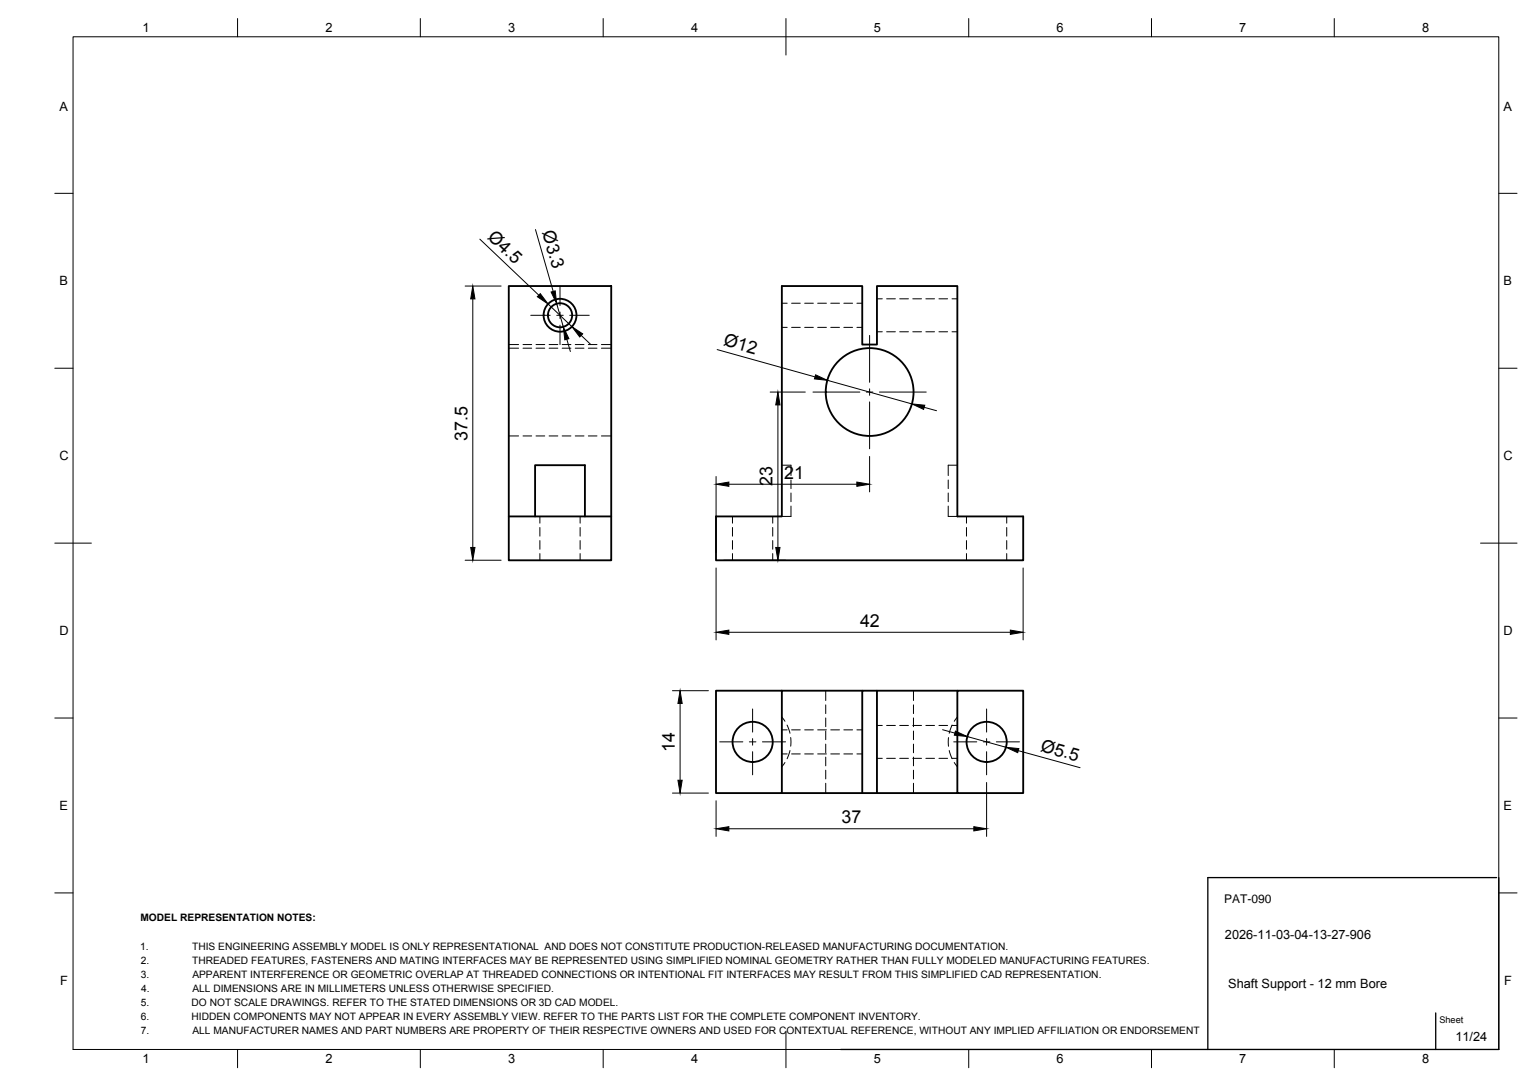
ISO-10303-21;
HEADER;
/* Generated by software containing ST-Developer
 * from STEP Tools, Inc. (www.steptools.com) 
 */

FILE_DESCRIPTION(
/* description */ ('Round-Shaft Linear Stage with Ball Bushings'),
/* implementation_level */ '2;1');

FILE_NAME(
/* name */ 'Shaft Support - 12 mm Bore.step',
/* time_stamp */ '2026-10-27T10:47:55-07:00',
/* author */ (''),
/* organization */ (''),
/* preprocessor_version */ 'ST-DEVELOPER v20.2',
/* originating_system */ 'Autodesk Translation Framework v15.17.0.0',
/* authorisation */ '');

FILE_SCHEMA (('AUTOMOTIVE_DESIGN { 1 0 10303 214 3 1 1 }'));
ENDSEC;

DATA;
#10=MECHANICAL_DESIGN_GEOMETRIC_PRESENTATION_REPRESENTATION('',(#308),#7835);
#266=SHAPE_REPRESENTATION_RELATIONSHIP('SRR','None',#7954,#287);
#287=ADVANCED_BREP_SHAPE_REPRESENTATION('',(#329),#7818);
#308=STYLED_ITEM('',(#8144),#329);
#329=MANIFOLD_SOLID_BREP('Body1',#4398);
#376=FACE_BOUND('',#973,.T.);
#377=FACE_BOUND('',#975,.T.);
#378=FACE_BOUND('',#977,.T.);
#379=FACE_BOUND('',#984,.T.);
#380=FACE_BOUND('',#987,.T.);
#381=FACE_BOUND('',#988,.T.);
#382=FACE_BOUND('',#991,.T.);
#383=FACE_BOUND('',#994,.T.);
#384=FACE_BOUND('',#997,.T.);
#385=FACE_BOUND('',#1000,.T.);
#495=PLANE('',#4761);
#496=PLANE('',#4768);
#497=PLANE('',#4769);
#498=PLANE('',#4771);
#499=PLANE('',#4773);
#500=PLANE('',#4787);
#501=PLANE('',#4788);
#502=PLANE('',#4789);
#503=PLANE('',#4790);
#504=PLANE('',#4791);
#505=PLANE('',#4792);
#506=PLANE('',#4793);
#507=PLANE('',#4794);
#508=PLANE('',#4795);
#509=PLANE('',#4796);
#510=PLANE('',#4797);
#675=FACE_OUTER_BOUND('',#968,.T.);
#676=FACE_OUTER_BOUND('',#969,.T.);
#677=FACE_OUTER_BOUND('',#970,.T.);
#678=FACE_OUTER_BOUND('',#971,.T.);
#679=FACE_OUTER_BOUND('',#972,.T.);
#680=FACE_OUTER_BOUND('',#974,.T.);
#681=FACE_OUTER_BOUND('',#976,.T.);
#682=FACE_OUTER_BOUND('',#978,.T.);
#683=FACE_OUTER_BOUND('',#979,.T.);
#684=FACE_OUTER_BOUND('',#980,.T.);
#685=FACE_OUTER_BOUND('',#981,.T.);
#686=FACE_OUTER_BOUND('',#982,.T.);
#687=FACE_OUTER_BOUND('',#983,.T.);
#688=FACE_OUTER_BOUND('',#985,.T.);
#689=FACE_OUTER_BOUND('',#986,.T.);
#690=FACE_OUTER_BOUND('',#989,.T.);
#691=FACE_OUTER_BOUND('',#990,.T.);
#692=FACE_OUTER_BOUND('',#992,.T.);
#693=FACE_OUTER_BOUND('',#993,.T.);
#694=FACE_OUTER_BOUND('',#995,.T.);
#695=FACE_OUTER_BOUND('',#996,.T.);
#696=FACE_OUTER_BOUND('',#998,.T.);
#697=FACE_OUTER_BOUND('',#999,.T.);
#968=EDGE_LOOP('',(#3248,#3249));
#969=EDGE_LOOP('',(#3250,#3251,#3252,#3253));
#970=EDGE_LOOP('',(#3254,#3255,#3256,#3257));
#971=EDGE_LOOP('',(#3258,#3259));
#972=EDGE_LOOP('',(#3260,#3261,#3262,#3263,#3264,#3265));
#973=EDGE_LOOP('',(#3266));
#974=EDGE_LOOP('',(#3267,#3268,#3269,#3270,#3271,#3272,#3273,#3274));
#975=EDGE_LOOP('',(#3275));
#976=EDGE_LOOP('',(#3276,#3277,#3278,#3279,#3280,#3281));
#977=EDGE_LOOP('',(#3282));
#978=EDGE_LOOP('',(#3283,#3284,#3285,#3286));
#979=EDGE_LOOP('',(#3287,#3288,#3289,#3290));
#980=EDGE_LOOP('',(#3291,#3292,#3293,#3294));
#981=EDGE_LOOP('',(#3295,#3296,#3297,#3298));
#982=EDGE_LOOP('',(#3299,#3300,#3301,#3302));
#983=EDGE_LOOP('',(#3303,#3304,#3305,#3306,#3307,#3308,#3309,#3310,#3311,
#3312,#3313,#3314));
#984=EDGE_LOOP('',(#3315));
#985=EDGE_LOOP('',(#3316,#3317,#3318,#3319));
#986=EDGE_LOOP('',(#3320,#3321,#3322,#3323));
#987=EDGE_LOOP('',(#3324));
#988=EDGE_LOOP('',(#3325));
#989=EDGE_LOOP('',(#3326,#3327,#3328,#3329));
#990=EDGE_LOOP('',(#3330,#3331,#3332,#3333,#3334,#3335,#3336,#3337));
#991=EDGE_LOOP('',(#3338));
#992=EDGE_LOOP('',(#3339,#3340,#3341,#3342));
#993=EDGE_LOOP('',(#3343,#3344,#3345,#3346));
#994=EDGE_LOOP('',(#3347));
#995=EDGE_LOOP('',(#3348,#3349,#3350,#3351));
#996=EDGE_LOOP('',(#3352,#3353,#3354,#3355));
#997=EDGE_LOOP('',(#3356));
#998=EDGE_LOOP('',(#3357,#3358,#3359,#3360));
#999=EDGE_LOOP('',(#3361,#3362,#3363,#3364,#3365,#3366,#3367,#3368,#3369,
#3370,#3371,#3372));
#1000=EDGE_LOOP('',(#3373));
#1332=LINE('',#6852,#1672);
#1333=LINE('',#6856,#1673);
#1334=LINE('',#6859,#1674);
#1335=LINE('',#6863,#1675);
#1336=LINE('',#6867,#1676);
#1337=LINE('',#6870,#1677);
#1338=LINE('',#6873,#1678);
#1339=LINE('',#6875,#1679);
#1340=LINE('',#6877,#1680);
#1341=LINE('',#6879,#1681);
#1342=LINE('',#6880,#1682);
#1343=LINE('',#6885,#1683);
#1344=LINE('',#6887,#1684);
#1345=LINE('',#6888,#1685);
#1346=LINE('',#6894,#1686);
#1347=LINE('',#6896,#1687);
#1348=LINE('',#6897,#1688);
#1349=LINE('',#6899,#1689);
#1350=LINE('',#6900,#1690);
#1351=LINE('',#6907,#1691);
#1352=LINE('',#6911,#1692);
#1353=LINE('',#6916,#1693);
#1354=LINE('',#6920,#1694);
#1355=LINE('',#6925,#1695);
#1356=LINE('',#6929,#1696);
#1357=LINE('',#6931,#1697);
#1358=LINE('',#6932,#1698);
#1359=LINE('',#6934,#1699);
#1360=LINE('',#6936,#1700);
#1361=LINE('',#6938,#1701);
#1362=LINE('',#6940,#1702);
#1363=LINE('',#6942,#1703);
#1364=LINE('',#6943,#1704);
#1365=LINE('',#6946,#1705);
#1366=LINE('',#6947,#1706);
#1367=LINE('',#6950,#1707);
#1368=LINE('',#6951,#1708);
#1369=LINE('',#6953,#1709);
#1370=LINE('',#6956,#1710);
#1371=LINE('',#6957,#1711);
#1372=LINE('',#6960,#1712);
#1373=LINE('',#6961,#1713);
#1374=LINE('',#6964,#1714);
#1375=LINE('',#6965,#1715);
#1376=LINE('',#6968,#1716);
#1377=LINE('',#6969,#1717);
#1378=LINE('',#6972,#1718);
#1379=LINE('',#6973,#1719);
#1380=LINE('',#6975,#1720);
#1672=VECTOR('',#5485,1.);
#1673=VECTOR('',#5490,1.);
#1674=VECTOR('',#5493,1.);
#1675=VECTOR('',#5496,1.);
#1676=VECTOR('',#5499,1.);
#1677=VECTOR('',#5504,1.);
#1678=VECTOR('',#5507,1.);
#1679=VECTOR('',#5508,1.);
#1680=VECTOR('',#5509,1.);
#1681=VECTOR('',#5510,1.);
#1682=VECTOR('',#5511,1.);
#1683=VECTOR('',#5516,1.);
#1684=VECTOR('',#5517,1.);
#1685=VECTOR('',#5518,1.);
#1686=VECTOR('',#5523,1.);
#1687=VECTOR('',#5524,1.);
#1688=VECTOR('',#5525,1.);
#1689=VECTOR('',#5526,1.);
#1690=VECTOR('',#5527,1.);
#1691=VECTOR('',#5534,0.225);
#1692=VECTOR('',#5539,0.165);
#1693=VECTOR('',#5546,0.275);
#1694=VECTOR('',#5551,0.275);
#1695=VECTOR('',#5556,0.6);
#1696=VECTOR('',#5561,1.);
#1697=VECTOR('',#5562,1.);
#1698=VECTOR('',#5563,1.);
#1699=VECTOR('',#5564,1.);
#1700=VECTOR('',#5565,1.);
#1701=VECTOR('',#5566,1.);
#1702=VECTOR('',#5567,1.);
#1703=VECTOR('',#5568,1.);
#1704=VECTOR('',#5569,1.);
#1705=VECTOR('',#5572,1.);
#1706=VECTOR('',#5573,1.);
#1707=VECTOR('',#5576,1.);
#1708=VECTOR('',#5577,1.);
#1709=VECTOR('',#5580,1.);
#1710=VECTOR('',#5583,1.);
#1711=VECTOR('',#5584,1.);
#1712=VECTOR('',#5587,1.);
#1713=VECTOR('',#5588,1.);
#1714=VECTOR('',#5591,1.);
#1715=VECTOR('',#5592,1.);
#1716=VECTOR('',#5595,1.);
#1717=VECTOR('',#5596,1.);
#1718=VECTOR('',#5599,1.);
#1719=VECTOR('',#5600,1.);
#1720=VECTOR('',#5603,1.);
#1973=CIRCLE('',#4762,0.525);
#1974=CIRCLE('',#4764,0.525);
#1975=CIRCLE('',#4766,0.525);
#1976=CIRCLE('',#4767,0.525);
#1977=CIRCLE('',#4770,0.275);
#1978=CIRCLE('',#4772,0.165);
#1979=CIRCLE('',#4774,0.275);
#1980=CIRCLE('',#4776,0.225);
#1981=CIRCLE('',#4777,0.225);
#1982=CIRCLE('',#4779,0.165);
#1983=CIRCLE('',#4781,0.275);
#1984=CIRCLE('',#4783,0.275);
#1985=CIRCLE('',#4785,0.6);
#1986=CIRCLE('',#4786,0.6);
#2202=VERTEX_POINT('',#6850);
#2203=VERTEX_POINT('',#6851);
#2204=VERTEX_POINT('',#6855);
#2205=VERTEX_POINT('',#6857);
#2206=VERTEX_POINT('',#6861);
#2207=VERTEX_POINT('',#6862);
#2208=VERTEX_POINT('',#6864);
#2209=VERTEX_POINT('',#6866);
#2210=VERTEX_POINT('',#6872);
#2211=VERTEX_POINT('',#6874);
#2212=VERTEX_POINT('',#6876);
#2213=VERTEX_POINT('',#6878);
#2214=VERTEX_POINT('',#6881);
#2215=VERTEX_POINT('',#6884);
#2216=VERTEX_POINT('',#6886);
#2217=VERTEX_POINT('',#6889);
#2218=VERTEX_POINT('',#6892);
#2219=VERTEX_POINT('',#6893);
#2220=VERTEX_POINT('',#6895);
#2221=VERTEX_POINT('',#6898);
#2222=VERTEX_POINT('',#6901);
#2223=VERTEX_POINT('',#6904);
#2224=VERTEX_POINT('',#6906);
#2225=VERTEX_POINT('',#6910);
#2226=VERTEX_POINT('',#6914);
#2227=VERTEX_POINT('',#6918);
#2228=VERTEX_POINT('',#6922);
#2229=VERTEX_POINT('',#6924);
#2230=VERTEX_POINT('',#6928);
#2231=VERTEX_POINT('',#6930);
#2232=VERTEX_POINT('',#6933);
#2233=VERTEX_POINT('',#6935);
#2234=VERTEX_POINT('',#6937);
#2235=VERTEX_POINT('',#6939);
#2236=VERTEX_POINT('',#6941);
#2237=VERTEX_POINT('',#6945);
#2238=VERTEX_POINT('',#6949);
#2239=VERTEX_POINT('',#6955);
#2240=VERTEX_POINT('',#6959);
#2241=VERTEX_POINT('',#6963);
#2242=VERTEX_POINT('',#6967);
#2243=VERTEX_POINT('',#6971);
#2592=EDGE_CURVE('',#2202,#2203,#1332,.T.);
#2593=EDGE_CURVE('',#2203,#2202,#1973,.T.);
#2594=EDGE_CURVE('',#2204,#2202,#1333,.T.);
#2595=EDGE_CURVE('',#2205,#2204,#1974,.T.);
#2596=EDGE_CURVE('',#2203,#2205,#1334,.T.);
#2597=EDGE_CURVE('',#2206,#2207,#1335,.T.);
#2598=EDGE_CURVE('',#2206,#2208,#1975,.T.);
#2599=EDGE_CURVE('',#2209,#2208,#1336,.T.);
#2600=EDGE_CURVE('',#2207,#2209,#1976,.T.);
#2601=EDGE_CURVE('',#2208,#2206,#1337,.T.);
#2602=EDGE_CURVE('',#2204,#2210,#1338,.T.);
#2603=EDGE_CURVE('',#2211,#2210,#1339,.T.);
#2604=EDGE_CURVE('',#2211,#2212,#1340,.T.);
#2605=EDGE_CURVE('',#2213,#2212,#1341,.T.);
#2606=EDGE_CURVE('',#2213,#2205,#1342,.T.);
#2607=EDGE_CURVE('',#2214,#2214,#1977,.T.);
#2608=EDGE_CURVE('',#2215,#2213,#1343,.T.);
#2609=EDGE_CURVE('',#2215,#2216,#1344,.T.);
#2610=EDGE_CURVE('',#2210,#2216,#1345,.T.);
#2611=EDGE_CURVE('',#2217,#2217,#1978,.T.);
#2612=EDGE_CURVE('',#2218,#2219,#1346,.T.);
#2613=EDGE_CURVE('',#2220,#2219,#1347,.T.);
#2614=EDGE_CURVE('',#2207,#2220,#1348,.T.);
#2615=EDGE_CURVE('',#2221,#2209,#1349,.T.);
#2616=EDGE_CURVE('',#2218,#2221,#1350,.T.);
#2617=EDGE_CURVE('',#2222,#2222,#1979,.T.);
#2618=EDGE_CURVE('',#2223,#2223,#1980,.T.);
#2619=EDGE_CURVE('',#2223,#2224,#1351,.T.);
#2620=EDGE_CURVE('',#2224,#2224,#1981,.T.);
#2621=EDGE_CURVE('',#2217,#2225,#1352,.T.);
#2622=EDGE_CURVE('',#2225,#2225,#1982,.T.);
#2623=EDGE_CURVE('',#2226,#2226,#1983,.T.);
#2624=EDGE_CURVE('',#2226,#2214,#1353,.T.);
#2625=EDGE_CURVE('',#2227,#2227,#1984,.T.);
#2626=EDGE_CURVE('',#2227,#2222,#1354,.T.);
#2627=EDGE_CURVE('',#2228,#2228,#1985,.T.);
#2628=EDGE_CURVE('',#2228,#2229,#1355,.T.);
#2629=EDGE_CURVE('',#2229,#2229,#1986,.T.);
#2630=EDGE_CURVE('',#2212,#2230,#1356,.T.);
#2631=EDGE_CURVE('',#2230,#2231,#1357,.T.);
#2632=EDGE_CURVE('',#2231,#2218,#1358,.T.);
#2633=EDGE_CURVE('',#2221,#2232,#1359,.T.);
#2634=EDGE_CURVE('',#2232,#2233,#1360,.T.);
#2635=EDGE_CURVE('',#2233,#2234,#1361,.T.);
#2636=EDGE_CURVE('',#2234,#2235,#1362,.T.);
#2637=EDGE_CURVE('',#2235,#2236,#1363,.T.);
#2638=EDGE_CURVE('',#2236,#2215,#1364,.T.);
#2639=EDGE_CURVE('',#2237,#2211,#1365,.T.);
#2640=EDGE_CURVE('',#2230,#2237,#1366,.T.);
#2641=EDGE_CURVE('',#2238,#2237,#1367,.T.);
#2642=EDGE_CURVE('',#2231,#2238,#1368,.T.);
#2643=EDGE_CURVE('',#2219,#2238,#1369,.T.);
#2644=EDGE_CURVE('',#2239,#2220,#1370,.T.);
#2645=EDGE_CURVE('',#2232,#2239,#1371,.T.);
#2646=EDGE_CURVE('',#2240,#2239,#1372,.T.);
#2647=EDGE_CURVE('',#2233,#2240,#1373,.T.);
#2648=EDGE_CURVE('',#2241,#2240,#1374,.T.);
#2649=EDGE_CURVE('',#2234,#2241,#1375,.T.);
#2650=EDGE_CURVE('',#2242,#2241,#1376,.T.);
#2651=EDGE_CURVE('',#2235,#2242,#1377,.T.);
#2652=EDGE_CURVE('',#2243,#2242,#1378,.T.);
#2653=EDGE_CURVE('',#2236,#2243,#1379,.T.);
#2654=EDGE_CURVE('',#2216,#2243,#1380,.T.);
#3248=ORIENTED_EDGE('',*,*,#2592,.F.);
#3249=ORIENTED_EDGE('',*,*,#2593,.F.);
#3250=ORIENTED_EDGE('',*,*,#2594,.F.);
#3251=ORIENTED_EDGE('',*,*,#2595,.F.);
#3252=ORIENTED_EDGE('',*,*,#2596,.F.);
#3253=ORIENTED_EDGE('',*,*,#2593,.T.);
#3254=ORIENTED_EDGE('',*,*,#2597,.F.);
#3255=ORIENTED_EDGE('',*,*,#2598,.T.);
#3256=ORIENTED_EDGE('',*,*,#2599,.F.);
#3257=ORIENTED_EDGE('',*,*,#2600,.F.);
#3258=ORIENTED_EDGE('',*,*,#2601,.F.);
#3259=ORIENTED_EDGE('',*,*,#2598,.F.);
#3260=ORIENTED_EDGE('',*,*,#2602,.T.);
#3261=ORIENTED_EDGE('',*,*,#2603,.F.);
#3262=ORIENTED_EDGE('',*,*,#2604,.T.);
#3263=ORIENTED_EDGE('',*,*,#2605,.F.);
#3264=ORIENTED_EDGE('',*,*,#2606,.T.);
#3265=ORIENTED_EDGE('',*,*,#2595,.T.);
#3266=ORIENTED_EDGE('',*,*,#2607,.T.);
#3267=ORIENTED_EDGE('',*,*,#2594,.T.);
#3268=ORIENTED_EDGE('',*,*,#2592,.T.);
#3269=ORIENTED_EDGE('',*,*,#2596,.T.);
#3270=ORIENTED_EDGE('',*,*,#2606,.F.);
#3271=ORIENTED_EDGE('',*,*,#2608,.F.);
#3272=ORIENTED_EDGE('',*,*,#2609,.T.);
#3273=ORIENTED_EDGE('',*,*,#2610,.F.);
#3274=ORIENTED_EDGE('',*,*,#2602,.F.);
#3275=ORIENTED_EDGE('',*,*,#2611,.T.);
#3276=ORIENTED_EDGE('',*,*,#2612,.T.);
#3277=ORIENTED_EDGE('',*,*,#2613,.F.);
#3278=ORIENTED_EDGE('',*,*,#2614,.F.);
#3279=ORIENTED_EDGE('',*,*,#2600,.T.);
#3280=ORIENTED_EDGE('',*,*,#2615,.F.);
#3281=ORIENTED_EDGE('',*,*,#2616,.F.);
#3282=ORIENTED_EDGE('',*,*,#2617,.T.);
#3283=ORIENTED_EDGE('',*,*,#2618,.F.);
#3284=ORIENTED_EDGE('',*,*,#2619,.T.);
#3285=ORIENTED_EDGE('',*,*,#2620,.F.);
#3286=ORIENTED_EDGE('',*,*,#2619,.F.);
#3287=ORIENTED_EDGE('',*,*,#2611,.F.);
#3288=ORIENTED_EDGE('',*,*,#2621,.T.);
#3289=ORIENTED_EDGE('',*,*,#2622,.F.);
#3290=ORIENTED_EDGE('',*,*,#2621,.F.);
#3291=ORIENTED_EDGE('',*,*,#2623,.F.);
#3292=ORIENTED_EDGE('',*,*,#2624,.T.);
#3293=ORIENTED_EDGE('',*,*,#2607,.F.);
#3294=ORIENTED_EDGE('',*,*,#2624,.F.);
#3295=ORIENTED_EDGE('',*,*,#2625,.F.);
#3296=ORIENTED_EDGE('',*,*,#2626,.T.);
#3297=ORIENTED_EDGE('',*,*,#2617,.F.);
#3298=ORIENTED_EDGE('',*,*,#2626,.F.);
#3299=ORIENTED_EDGE('',*,*,#2627,.F.);
#3300=ORIENTED_EDGE('',*,*,#2628,.T.);
#3301=ORIENTED_EDGE('',*,*,#2629,.F.);
#3302=ORIENTED_EDGE('',*,*,#2628,.F.);
#3303=ORIENTED_EDGE('',*,*,#2605,.T.);
#3304=ORIENTED_EDGE('',*,*,#2630,.T.);
#3305=ORIENTED_EDGE('',*,*,#2631,.T.);
#3306=ORIENTED_EDGE('',*,*,#2632,.T.);
#3307=ORIENTED_EDGE('',*,*,#2616,.T.);
#3308=ORIENTED_EDGE('',*,*,#2633,.T.);
#3309=ORIENTED_EDGE('',*,*,#2634,.T.);
#3310=ORIENTED_EDGE('',*,*,#2635,.T.);
#3311=ORIENTED_EDGE('',*,*,#2636,.T.);
#3312=ORIENTED_EDGE('',*,*,#2637,.T.);
#3313=ORIENTED_EDGE('',*,*,#2638,.T.);
#3314=ORIENTED_EDGE('',*,*,#2608,.T.);
#3315=ORIENTED_EDGE('',*,*,#2627,.T.);
#3316=ORIENTED_EDGE('',*,*,#2604,.F.);
#3317=ORIENTED_EDGE('',*,*,#2639,.F.);
#3318=ORIENTED_EDGE('',*,*,#2640,.F.);
#3319=ORIENTED_EDGE('',*,*,#2630,.F.);
#3320=ORIENTED_EDGE('',*,*,#2640,.T.);
#3321=ORIENTED_EDGE('',*,*,#2641,.F.);
#3322=ORIENTED_EDGE('',*,*,#2642,.F.);
#3323=ORIENTED_EDGE('',*,*,#2631,.F.);
#3324=ORIENTED_EDGE('',*,*,#2623,.T.);
#3325=ORIENTED_EDGE('',*,*,#2625,.T.);
#3326=ORIENTED_EDGE('',*,*,#2642,.T.);
#3327=ORIENTED_EDGE('',*,*,#2643,.F.);
#3328=ORIENTED_EDGE('',*,*,#2612,.F.);
#3329=ORIENTED_EDGE('',*,*,#2632,.F.);
#3330=ORIENTED_EDGE('',*,*,#2597,.T.);
#3331=ORIENTED_EDGE('',*,*,#2614,.T.);
#3332=ORIENTED_EDGE('',*,*,#2644,.F.);
#3333=ORIENTED_EDGE('',*,*,#2645,.F.);
#3334=ORIENTED_EDGE('',*,*,#2633,.F.);
#3335=ORIENTED_EDGE('',*,*,#2615,.T.);
#3336=ORIENTED_EDGE('',*,*,#2599,.T.);
#3337=ORIENTED_EDGE('',*,*,#2601,.T.);
#3338=ORIENTED_EDGE('',*,*,#2620,.T.);
#3339=ORIENTED_EDGE('',*,*,#2645,.T.);
#3340=ORIENTED_EDGE('',*,*,#2646,.F.);
#3341=ORIENTED_EDGE('',*,*,#2647,.F.);
#3342=ORIENTED_EDGE('',*,*,#2634,.F.);
#3343=ORIENTED_EDGE('',*,*,#2647,.T.);
#3344=ORIENTED_EDGE('',*,*,#2648,.F.);
#3345=ORIENTED_EDGE('',*,*,#2649,.F.);
#3346=ORIENTED_EDGE('',*,*,#2635,.F.);
#3347=ORIENTED_EDGE('',*,*,#2618,.T.);
#3348=ORIENTED_EDGE('',*,*,#2649,.T.);
#3349=ORIENTED_EDGE('',*,*,#2650,.F.);
#3350=ORIENTED_EDGE('',*,*,#2651,.F.);
#3351=ORIENTED_EDGE('',*,*,#2636,.F.);
#3352=ORIENTED_EDGE('',*,*,#2651,.T.);
#3353=ORIENTED_EDGE('',*,*,#2652,.F.);
#3354=ORIENTED_EDGE('',*,*,#2653,.F.);
#3355=ORIENTED_EDGE('',*,*,#2637,.F.);
#3356=ORIENTED_EDGE('',*,*,#2622,.T.);
#3357=ORIENTED_EDGE('',*,*,#2653,.T.);
#3358=ORIENTED_EDGE('',*,*,#2654,.F.);
#3359=ORIENTED_EDGE('',*,*,#2609,.F.);
#3360=ORIENTED_EDGE('',*,*,#2638,.F.);
#3361=ORIENTED_EDGE('',*,*,#2603,.T.);
#3362=ORIENTED_EDGE('',*,*,#2610,.T.);
#3363=ORIENTED_EDGE('',*,*,#2654,.T.);
#3364=ORIENTED_EDGE('',*,*,#2652,.T.);
#3365=ORIENTED_EDGE('',*,*,#2650,.T.);
#3366=ORIENTED_EDGE('',*,*,#2648,.T.);
#3367=ORIENTED_EDGE('',*,*,#2646,.T.);
#3368=ORIENTED_EDGE('',*,*,#2644,.T.);
#3369=ORIENTED_EDGE('',*,*,#2613,.T.);
#3370=ORIENTED_EDGE('',*,*,#2643,.T.);
#3371=ORIENTED_EDGE('',*,*,#2641,.T.);
#3372=ORIENTED_EDGE('',*,*,#2639,.T.);
#3373=ORIENTED_EDGE('',*,*,#2629,.T.);
#4073=CYLINDRICAL_SURFACE('',#4763,0.525);
#4074=CYLINDRICAL_SURFACE('',#4765,0.525);
#4075=CYLINDRICAL_SURFACE('',#4775,0.225);
#4076=CYLINDRICAL_SURFACE('',#4778,0.165);
#4077=CYLINDRICAL_SURFACE('',#4780,0.275);
#4078=CYLINDRICAL_SURFACE('',#4782,0.275);
#4079=CYLINDRICAL_SURFACE('',#4784,0.6);
#4194=ADVANCED_FACE('',(#675),#495,.F.);
#4195=ADVANCED_FACE('',(#676),#4073,.F.);
#4196=ADVANCED_FACE('',(#677),#4074,.F.);
#4197=ADVANCED_FACE('',(#678),#496,.F.);
#4198=ADVANCED_FACE('',(#679,#376),#497,.T.);
#4199=ADVANCED_FACE('',(#680,#377),#498,.T.);
#4200=ADVANCED_FACE('',(#681,#378),#499,.T.);
#4201=ADVANCED_FACE('',(#682),#4075,.F.);
#4202=ADVANCED_FACE('',(#683),#4076,.F.);
#4203=ADVANCED_FACE('',(#684),#4077,.F.);
#4204=ADVANCED_FACE('',(#685),#4078,.F.);
#4205=ADVANCED_FACE('',(#686),#4079,.F.);
#4206=ADVANCED_FACE('',(#687,#379),#500,.T.);
#4207=ADVANCED_FACE('',(#688),#501,.T.);
#4208=ADVANCED_FACE('',(#689,#380,#381),#502,.T.);
#4209=ADVANCED_FACE('',(#690),#503,.T.);
#4210=ADVANCED_FACE('',(#691,#382),#504,.T.);
#4211=ADVANCED_FACE('',(#692),#505,.T.);
#4212=ADVANCED_FACE('',(#693,#383),#506,.T.);
#4213=ADVANCED_FACE('',(#694),#507,.T.);
#4214=ADVANCED_FACE('',(#695,#384),#508,.T.);
#4215=ADVANCED_FACE('',(#696),#509,.T.);
#4216=ADVANCED_FACE('',(#697,#385),#510,.T.);
#4398=CLOSED_SHELL('',(#4194,#4195,#4196,#4197,#4198,#4199,#4200,#4201,
#4202,#4203,#4204,#4205,#4206,#4207,#4208,#4209,#4210,#4211,#4212,#4213,
#4214,#4215,#4216));
#4760=AXIS2_PLACEMENT_3D('',#6848,#5481,#5482);
#4761=AXIS2_PLACEMENT_3D('',#6849,#5483,#5484);
#4762=AXIS2_PLACEMENT_3D('',#6853,#5486,#5487);
#4763=AXIS2_PLACEMENT_3D('',#6854,#5488,#5489);
#4764=AXIS2_PLACEMENT_3D('',#6858,#5491,#5492);
#4765=AXIS2_PLACEMENT_3D('',#6860,#5494,#5495);
#4766=AXIS2_PLACEMENT_3D('',#6865,#5497,#5498);
#4767=AXIS2_PLACEMENT_3D('',#6868,#5500,#5501);
#4768=AXIS2_PLACEMENT_3D('',#6869,#5502,#5503);
#4769=AXIS2_PLACEMENT_3D('',#6871,#5505,#5506);
#4770=AXIS2_PLACEMENT_3D('',#6882,#5512,#5513);
#4771=AXIS2_PLACEMENT_3D('',#6883,#5514,#5515);
#4772=AXIS2_PLACEMENT_3D('',#6890,#5519,#5520);
#4773=AXIS2_PLACEMENT_3D('',#6891,#5521,#5522);
#4774=AXIS2_PLACEMENT_3D('',#6902,#5528,#5529);
#4775=AXIS2_PLACEMENT_3D('',#6903,#5530,#5531);
#4776=AXIS2_PLACEMENT_3D('',#6905,#5532,#5533);
#4777=AXIS2_PLACEMENT_3D('',#6908,#5535,#5536);
#4778=AXIS2_PLACEMENT_3D('',#6909,#5537,#5538);
#4779=AXIS2_PLACEMENT_3D('',#6912,#5540,#5541);
#4780=AXIS2_PLACEMENT_3D('',#6913,#5542,#5543);
#4781=AXIS2_PLACEMENT_3D('',#6915,#5544,#5545);
#4782=AXIS2_PLACEMENT_3D('',#6917,#5547,#5548);
#4783=AXIS2_PLACEMENT_3D('',#6919,#5549,#5550);
#4784=AXIS2_PLACEMENT_3D('',#6921,#5552,#5553);
#4785=AXIS2_PLACEMENT_3D('',#6923,#5554,#5555);
#4786=AXIS2_PLACEMENT_3D('',#6926,#5557,#5558);
#4787=AXIS2_PLACEMENT_3D('',#6927,#5559,#5560);
#4788=AXIS2_PLACEMENT_3D('',#6944,#5570,#5571);
#4789=AXIS2_PLACEMENT_3D('',#6948,#5574,#5575);
#4790=AXIS2_PLACEMENT_3D('',#6952,#5578,#5579);
#4791=AXIS2_PLACEMENT_3D('',#6954,#5581,#5582);
#4792=AXIS2_PLACEMENT_3D('',#6958,#5585,#5586);
#4793=AXIS2_PLACEMENT_3D('',#6962,#5589,#5590);
#4794=AXIS2_PLACEMENT_3D('',#6966,#5593,#5594);
#4795=AXIS2_PLACEMENT_3D('',#6970,#5597,#5598);
#4796=AXIS2_PLACEMENT_3D('',#6974,#5601,#5602);
#4797=AXIS2_PLACEMENT_3D('',#6976,#5604,#5605);
#5481=DIRECTION('axis',(0.,0.,1.));
#5482=DIRECTION('refdir',(1.,0.,0.));
#5483=DIRECTION('center_axis',(0.,0.,1.));
#5484=DIRECTION('ref_axis',(1.,0.,0.));
#5485=DIRECTION('',(0.,-1.,0.));
#5486=DIRECTION('center_axis',(0.,0.,1.));
#5487=DIRECTION('ref_axis',(1.,0.,0.));
#5488=DIRECTION('center_axis',(0.,0.,1.));
#5489=DIRECTION('ref_axis',(1.,0.,0.));
#5490=DIRECTION('',(0.,0.,1.));
#5491=DIRECTION('center_axis',(0.,0.,1.));
#5492=DIRECTION('ref_axis',(1.,0.,0.));
#5493=DIRECTION('',(0.,0.,-1.));
#5494=DIRECTION('center_axis',(0.,0.,1.));
#5495=DIRECTION('ref_axis',(-1.,1.22464679914735E-16,0.));
#5496=DIRECTION('',(0.,0.,-1.));
#5497=DIRECTION('center_axis',(0.,0.,1.));
#5498=DIRECTION('ref_axis',(1.,0.,0.));
#5499=DIRECTION('',(0.,0.,1.));
#5500=DIRECTION('center_axis',(0.,0.,1.));
#5501=DIRECTION('ref_axis',(1.,0.,0.));
#5502=DIRECTION('center_axis',(0.,0.,1.));
#5503=DIRECTION('ref_axis',(1.,0.,0.));
#5504=DIRECTION('',(0.,1.,0.));
#5505=DIRECTION('center_axis',(0.,0.,1.));
#5506=DIRECTION('ref_axis',(1.,0.,0.));
#5507=DIRECTION('',(0.,1.,0.));
#5508=DIRECTION('',(1.,0.,0.));
#5509=DIRECTION('',(0.,-1.,0.));
#5510=DIRECTION('',(-1.,0.,0.));
#5511=DIRECTION('',(0.,1.,0.));
#5512=DIRECTION('center_axis',(0.,0.,-1.));
#5513=DIRECTION('ref_axis',(1.,0.,0.));
#5514=DIRECTION('center_axis',(-1.,0.,0.));
#5515=DIRECTION('ref_axis',(0.,0.,1.));
#5516=DIRECTION('',(0.,0.,-1.));
#5517=DIRECTION('',(0.,1.,0.));
#5518=DIRECTION('',(0.,0.,1.));
#5519=DIRECTION('center_axis',(1.,0.,0.));
#5520=DIRECTION('ref_axis',(0.,0.,-1.));
#5521=DIRECTION('center_axis',(0.,0.,1.));
#5522=DIRECTION('ref_axis',(1.,0.,0.));
#5523=DIRECTION('',(0.,1.,0.));
#5524=DIRECTION('',(1.,0.,0.));
#5525=DIRECTION('',(0.,1.,0.));
#5526=DIRECTION('',(0.,1.,0.));
#5527=DIRECTION('',(-1.,0.,0.));
#5528=DIRECTION('center_axis',(0.,0.,-1.));
#5529=DIRECTION('ref_axis',(1.,0.,0.));
#5530=DIRECTION('center_axis',(1.,0.,0.));
#5531=DIRECTION('ref_axis',(0.,0.,-1.));
#5532=DIRECTION('center_axis',(1.,0.,0.));
#5533=DIRECTION('ref_axis',(0.,0.,-1.));
#5534=DIRECTION('',(1.,0.,0.));
#5535=DIRECTION('center_axis',(-1.,0.,0.));
#5536=DIRECTION('ref_axis',(0.,0.,-1.));
#5537=DIRECTION('center_axis',(1.,0.,0.));
#5538=DIRECTION('ref_axis',(0.,0.,-1.));
#5539=DIRECTION('',(1.,0.,0.));
#5540=DIRECTION('center_axis',(-1.,0.,0.));
#5541=DIRECTION('ref_axis',(0.,0.,-1.));
#5542=DIRECTION('center_axis',(0.,0.,1.));
#5543=DIRECTION('ref_axis',(1.,0.,0.));
#5544=DIRECTION('center_axis',(0.,0.,1.));
#5545=DIRECTION('ref_axis',(1.,0.,0.));
#5546=DIRECTION('',(0.,0.,1.));
#5547=DIRECTION('center_axis',(0.,0.,1.));
#5548=DIRECTION('ref_axis',(1.,0.,0.));
#5549=DIRECTION('center_axis',(0.,0.,1.));
#5550=DIRECTION('ref_axis',(1.,0.,0.));
#5551=DIRECTION('',(0.,0.,1.));
#5552=DIRECTION('center_axis',(0.,1.,0.));
#5553=DIRECTION('ref_axis',(1.,0.,0.));
#5554=DIRECTION('center_axis',(0.,1.,0.));
#5555=DIRECTION('ref_axis',(1.,0.,0.));
#5556=DIRECTION('',(0.,1.,0.));
#5557=DIRECTION('center_axis',(0.,-1.,0.));
#5558=DIRECTION('ref_axis',(1.,0.,0.));
#5559=DIRECTION('center_axis',(0.,-1.,0.));
#5560=DIRECTION('ref_axis',(0.,0.,-1.));
#5561=DIRECTION('',(0.,0.,-1.));
#5562=DIRECTION('',(1.,0.,0.));
#5563=DIRECTION('',(0.,0.,1.));
#5564=DIRECTION('',(0.,0.,1.));
#5565=DIRECTION('',(-1.,0.,0.));
#5566=DIRECTION('',(0.,0.,-1.));
#5567=DIRECTION('',(-1.,0.,0.));
#5568=DIRECTION('',(0.,0.,1.));
#5569=DIRECTION('',(-1.,0.,0.));
#5570=DIRECTION('center_axis',(-1.,0.,0.));
#5571=DIRECTION('ref_axis',(0.,0.,1.));
#5572=DIRECTION('',(0.,0.,1.));
#5573=DIRECTION('',(0.,1.,0.));
#5574=DIRECTION('center_axis',(0.,0.,-1.));
#5575=DIRECTION('ref_axis',(-1.,0.,0.));
#5576=DIRECTION('',(-1.,0.,0.));
#5577=DIRECTION('',(0.,1.,0.));
#5578=DIRECTION('center_axis',(1.,0.,0.));
#5579=DIRECTION('ref_axis',(0.,0.,-1.));
#5580=DIRECTION('',(0.,0.,-1.));
#5581=DIRECTION('center_axis',(1.,0.,0.));
#5582=DIRECTION('ref_axis',(0.,0.,-1.));
#5583=DIRECTION('',(0.,0.,-1.));
#5584=DIRECTION('',(0.,1.,0.));
#5585=DIRECTION('center_axis',(0.,0.,1.));
#5586=DIRECTION('ref_axis',(1.,0.,0.));
#5587=DIRECTION('',(1.,0.,0.));
#5588=DIRECTION('',(0.,1.,0.));
#5589=DIRECTION('center_axis',(-1.,0.,0.));
#5590=DIRECTION('ref_axis',(0.,0.,1.));
#5591=DIRECTION('',(0.,0.,1.));
#5592=DIRECTION('',(0.,1.,0.));
#5593=DIRECTION('center_axis',(0.,0.,1.));
#5594=DIRECTION('ref_axis',(1.,0.,0.));
#5595=DIRECTION('',(1.,0.,0.));
#5596=DIRECTION('',(0.,1.,0.));
#5597=DIRECTION('center_axis',(1.,0.,0.));
#5598=DIRECTION('ref_axis',(0.,0.,-1.));
#5599=DIRECTION('',(0.,0.,-1.));
#5600=DIRECTION('',(0.,1.,0.));
#5601=DIRECTION('center_axis',(0.,0.,1.));
#5602=DIRECTION('ref_axis',(1.,0.,0.));
#5603=DIRECTION('',(1.,0.,0.));
#5604=DIRECTION('center_axis',(0.,1.,0.));
#5605=DIRECTION('ref_axis',(0.,0.,1.));
#6848=CARTESIAN_POINT('',(0.,0.,0.));
#6849=CARTESIAN_POINT('Origin',(-1.6,0.,1.3));
#6850=CARTESIAN_POINT('',(-1.2,0.340036762718386,1.3));
#6851=CARTESIAN_POINT('',(-1.2,-0.340036762718386,1.3));
#6852=CARTESIAN_POINT('',(-1.2,0.,1.3));
#6853=CARTESIAN_POINT('Origin',(-1.6,0.,1.3));
#6854=CARTESIAN_POINT('Origin',(-1.6,0.,0.6));
#6855=CARTESIAN_POINT('',(-1.2,0.340036762718386,0.6));
#6856=CARTESIAN_POINT('',(-1.2,0.340036762718386,0.6));
#6857=CARTESIAN_POINT('',(-1.2,-0.340036762718386,0.6));
#6858=CARTESIAN_POINT('Origin',(-1.6,0.,0.6));
#6859=CARTESIAN_POINT('',(-1.2,-0.340036762718386,0.6));
#6860=CARTESIAN_POINT('Origin',(1.6,0.,0.6));
#6861=CARTESIAN_POINT('',(1.2,0.340036762718386,1.3));
#6862=CARTESIAN_POINT('',(1.2,0.340036762718386,0.6));
#6863=CARTESIAN_POINT('',(1.2,0.340036762718386,0.6));
#6864=CARTESIAN_POINT('',(1.2,-0.340036762718386,1.3));
#6865=CARTESIAN_POINT('Origin',(1.6,0.,1.3));
#6866=CARTESIAN_POINT('',(1.2,-0.340036762718386,0.6));
#6867=CARTESIAN_POINT('',(1.2,-0.340036762718386,0.6));
#6868=CARTESIAN_POINT('Origin',(1.6,0.,0.6));
#6869=CARTESIAN_POINT('Origin',(1.6,0.,1.3));
#6870=CARTESIAN_POINT('',(1.2,0.,1.3));
#6871=CARTESIAN_POINT('Origin',(-2.1,0.,0.6));
#6872=CARTESIAN_POINT('',(-1.2,0.7,0.6));
#6873=CARTESIAN_POINT('',(-1.2,0.,0.6));
#6874=CARTESIAN_POINT('',(-2.1,0.7,0.6));
#6875=CARTESIAN_POINT('',(-1.2,0.7,0.6));
#6876=CARTESIAN_POINT('',(-2.1,-0.7,0.6));
#6877=CARTESIAN_POINT('',(-2.1,0.,0.6));
#6878=CARTESIAN_POINT('',(-1.2,-0.7,0.6));
#6879=CARTESIAN_POINT('',(-1.2,-0.7,0.6));
#6880=CARTESIAN_POINT('',(-1.2,0.,0.6));
#6881=CARTESIAN_POINT('',(-1.875,3.36777869765522E-17,0.6));
#6882=CARTESIAN_POINT('Origin',(-1.6,0.,0.6));
#6883=CARTESIAN_POINT('Origin',(-1.2,0.,0.6));
#6884=CARTESIAN_POINT('',(-1.2,-0.7,3.75));
#6885=CARTESIAN_POINT('',(-1.2,-0.7,3.75));
#6886=CARTESIAN_POINT('',(-1.2,0.7,3.75));
#6887=CARTESIAN_POINT('',(-1.2,0.,3.75));
#6888=CARTESIAN_POINT('',(-1.2,0.7,3.75));
#6889=CARTESIAN_POINT('',(-1.2,-2.02066721859313E-17,3.515));
#6890=CARTESIAN_POINT('Origin',(-1.2,0.,3.35));
#6891=CARTESIAN_POINT('Origin',(1.2,0.,0.6));
#6892=CARTESIAN_POINT('',(2.1,-0.7,0.6));
#6893=CARTESIAN_POINT('',(2.1,0.7,0.6));
#6894=CARTESIAN_POINT('',(2.1,0.,0.6));
#6895=CARTESIAN_POINT('',(1.2,0.7,0.6));
#6896=CARTESIAN_POINT('',(2.1,0.7,0.6));
#6897=CARTESIAN_POINT('',(1.2,0.,0.6));
#6898=CARTESIAN_POINT('',(1.2,-0.7,0.6));
#6899=CARTESIAN_POINT('',(1.2,0.,0.6));
#6900=CARTESIAN_POINT('',(2.1,-0.7,0.6));
#6901=CARTESIAN_POINT('',(1.325,3.36777869765522E-17,0.6));
#6902=CARTESIAN_POINT('Origin',(1.6,0.,0.6));
#6903=CARTESIAN_POINT('Origin',(0.1,0.,3.35));
#6904=CARTESIAN_POINT('',(0.1,-2.75545529808155E-17,3.575));
#6905=CARTESIAN_POINT('Origin',(0.1,0.,3.35));
#6906=CARTESIAN_POINT('',(1.2,2.75545529808155E-17,3.575));
#6907=CARTESIAN_POINT('',(0.1,-2.75545529808155E-17,3.575));
#6908=CARTESIAN_POINT('Origin',(1.2,0.,3.35));
#6909=CARTESIAN_POINT('Origin',(0.,0.,3.35));
#6910=CARTESIAN_POINT('',(-0.1,2.02066721859313E-17,3.515));
#6911=CARTESIAN_POINT('',(0.,-2.02066721859313E-17,3.515));
#6912=CARTESIAN_POINT('Origin',(-0.1,0.,3.35));
#6913=CARTESIAN_POINT('Origin',(-1.6,0.,-0.05));
#6914=CARTESIAN_POINT('',(-1.875,-3.36777869765522E-17,0.));
#6915=CARTESIAN_POINT('Origin',(-1.6,0.,0.));
#6916=CARTESIAN_POINT('',(-1.875,-3.36777869765522E-17,-0.05));
#6917=CARTESIAN_POINT('Origin',(1.6,0.,-0.05));
#6918=CARTESIAN_POINT('',(1.325,-3.36777869765522E-17,0.));
#6919=CARTESIAN_POINT('Origin',(1.6,0.,0.));
#6920=CARTESIAN_POINT('',(1.325,-3.36777869765522E-17,-0.05));
#6921=CARTESIAN_POINT('Origin',(0.,0.,2.3));
#6922=CARTESIAN_POINT('',(-0.6,-0.7,2.3));
#6923=CARTESIAN_POINT('Origin',(0.,-0.7,2.3));
#6924=CARTESIAN_POINT('',(-0.6,0.7,2.3));
#6925=CARTESIAN_POINT('',(-0.6,0.,2.3));
#6926=CARTESIAN_POINT('Origin',(0.,0.7,2.3));
#6927=CARTESIAN_POINT('Origin',(0.,-0.7,1.875));
#6928=CARTESIAN_POINT('',(-2.1,-0.7,0.));
#6929=CARTESIAN_POINT('',(-2.1,-0.7,0.6));
#6930=CARTESIAN_POINT('',(2.1,-0.7,0.));
#6931=CARTESIAN_POINT('',(-2.1,-0.7,0.));
#6932=CARTESIAN_POINT('',(2.1,-0.7,0.));
#6933=CARTESIAN_POINT('',(1.2,-0.7,3.75));
#6934=CARTESIAN_POINT('',(1.2,-0.7,0.6));
#6935=CARTESIAN_POINT('',(0.1,-0.7,3.75));
#6936=CARTESIAN_POINT('',(1.2,-0.7,3.75));
#6937=CARTESIAN_POINT('',(0.1,-0.7,2.95));
#6938=CARTESIAN_POINT('',(0.1,-0.7,3.75));
#6939=CARTESIAN_POINT('',(-0.1,-0.7,2.95));
#6940=CARTESIAN_POINT('',(0.1,-0.7,2.95));
#6941=CARTESIAN_POINT('',(-0.1,-0.7,3.75));
#6942=CARTESIAN_POINT('',(-0.1,-0.7,2.95));
#6943=CARTESIAN_POINT('',(-0.1,-0.7,3.75));
#6944=CARTESIAN_POINT('Origin',(-2.1,0.,0.));
#6945=CARTESIAN_POINT('',(-2.1,0.7,0.));
#6946=CARTESIAN_POINT('',(-2.1,0.7,0.6));
#6947=CARTESIAN_POINT('',(-2.1,0.,0.));
#6948=CARTESIAN_POINT('Origin',(2.1,0.,0.));
#6949=CARTESIAN_POINT('',(2.1,0.7,0.));
#6950=CARTESIAN_POINT('',(-2.1,0.7,0.));
#6951=CARTESIAN_POINT('',(2.1,0.,0.));
#6952=CARTESIAN_POINT('Origin',(2.1,0.,0.6));
#6953=CARTESIAN_POINT('',(2.1,0.7,0.));
#6954=CARTESIAN_POINT('Origin',(1.2,0.,3.75));
#6955=CARTESIAN_POINT('',(1.2,0.7,3.75));
#6956=CARTESIAN_POINT('',(1.2,0.7,0.6));
#6957=CARTESIAN_POINT('',(1.2,0.,3.75));
#6958=CARTESIAN_POINT('Origin',(0.1,0.,3.75));
#6959=CARTESIAN_POINT('',(0.1,0.7,3.75));
#6960=CARTESIAN_POINT('',(1.2,0.7,3.75));
#6961=CARTESIAN_POINT('',(0.1,0.,3.75));
#6962=CARTESIAN_POINT('Origin',(0.1,0.,2.95));
#6963=CARTESIAN_POINT('',(0.1,0.7,2.95));
#6964=CARTESIAN_POINT('',(0.1,0.7,3.75));
#6965=CARTESIAN_POINT('',(0.1,0.,2.95));
#6966=CARTESIAN_POINT('Origin',(-0.1,0.,2.95));
#6967=CARTESIAN_POINT('',(-0.1,0.7,2.95));
#6968=CARTESIAN_POINT('',(0.1,0.7,2.95));
#6969=CARTESIAN_POINT('',(-0.1,0.,2.95));
#6970=CARTESIAN_POINT('Origin',(-0.1,0.,3.75));
#6971=CARTESIAN_POINT('',(-0.1,0.7,3.75));
#6972=CARTESIAN_POINT('',(-0.1,0.7,2.95));
#6973=CARTESIAN_POINT('',(-0.1,0.,3.75));
#6974=CARTESIAN_POINT('Origin',(-1.2,0.,3.75));
#6975=CARTESIAN_POINT('',(-0.1,0.7,3.75));
#6976=CARTESIAN_POINT('Origin',(0.,0.7,1.875));
#7792=UNCERTAINTY_MEASURE_WITH_UNIT(LENGTH_MEASURE(0.001),#7836,
'DISTANCE_ACCURACY_VALUE',
'Maximum model space distance between geometric entities at asserted c
onnectivities');
#7809=UNCERTAINTY_MEASURE_WITH_UNIT(LENGTH_MEASURE(0.001),#7836,
'DISTANCE_ACCURACY_VALUE',
'Maximum model space distance between geometric entities at asserted c
onnectivities');
#7818=(
GEOMETRIC_REPRESENTATION_CONTEXT(3)
GLOBAL_UNCERTAINTY_ASSIGNED_CONTEXT((#7792))
GLOBAL_UNIT_ASSIGNED_CONTEXT((#7836,#7838,#7839))
REPRESENTATION_CONTEXT('','3D')
);
#7835=(
GEOMETRIC_REPRESENTATION_CONTEXT(3)
GLOBAL_UNCERTAINTY_ASSIGNED_CONTEXT((#7809))
GLOBAL_UNIT_ASSIGNED_CONTEXT((#7836,#7838,#7839))
REPRESENTATION_CONTEXT('','3D')
);
#7836=(
LENGTH_UNIT()
NAMED_UNIT(*)
SI_UNIT(.CENTI.,.METRE.)
);
#7838=(
NAMED_UNIT(*)
PLANE_ANGLE_UNIT()
SI_UNIT($,.RADIAN.)
);
#7839=(
NAMED_UNIT(*)
SI_UNIT($,.STERADIAN.)
SOLID_ANGLE_UNIT()
);
#7848=SHAPE_DEFINITION_REPRESENTATION(#7873,#7954);
#7873=PRODUCT_DEFINITION_SHAPE('',$,#7980);
#7954=SHAPE_REPRESENTATION('',(#4760),#7818);
#7971=PRODUCT_DEFINITION_CONTEXT('part definition',#8048,'design');
#7980=PRODUCT_DEFINITION('Shaft Support - 12 mm Bore',
'Shaft Support - 12 mm Bore',#8005,#7971);
#8005=PRODUCT_DEFINITION_FORMATION('',$,#8058);
#8048=APPLICATION_CONTEXT(
'Core Data for Automotive Mechanical Design Process');
#8049=PRODUCT_CONTEXT('part definition',#8048,'mechanical');
#8058=PRODUCT('Shaft Support - 12 mm Bore','Shaft Support - 12 mm Bore',
'Shaft Support - 12 mm Bore',(#8049));
#8138=COLOUR_RGB('Grey',0.48,0.52,0.57);
#8139=FILL_AREA_STYLE_COLOUR('',#8138);
#8140=FILL_AREA_STYLE('',(#8139));
#8141=SURFACE_STYLE_FILL_AREA(#8140);
#8142=SURFACE_SIDE_STYLE('',(#8141));
#8143=SURFACE_STYLE_USAGE(.BOTH.,#8142);
#8144=PRESENTATION_STYLE_ASSIGNMENT((#8143));
ENDSEC;
END-ISO-10303-21;
